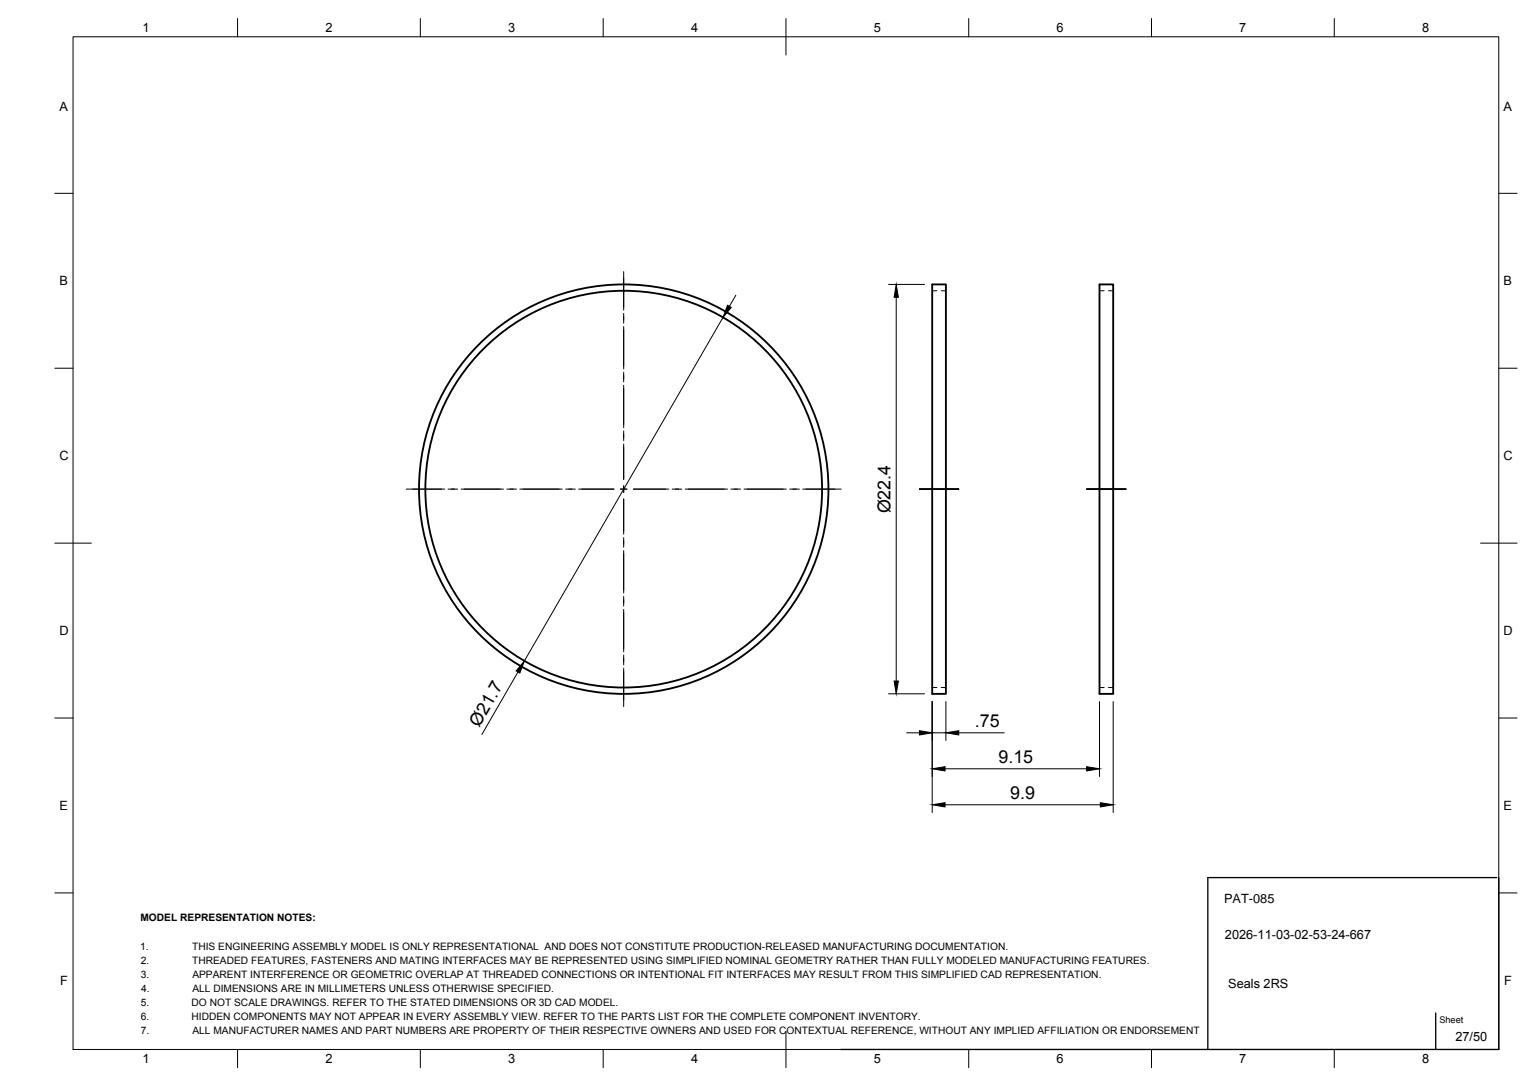
ISO-10303-21;
HEADER;
/* Generated by software containing ST-Developer
 * from STEP Tools, Inc. (www.steptools.com) 
 */

FILE_DESCRIPTION(
/* description */ ('Rack and pinion manual slide'),
/* implementation_level */ '2;1');

FILE_NAME(
/* name */ 'Seals 2RS.step',
/* time_stamp */ '2026-10-28T03:22:49-07:00',
/* author */ (''),
/* organization */ (''),
/* preprocessor_version */ 'ST-DEVELOPER v20.2',
/* originating_system */ 'Autodesk Translation Framework v15.17.0.0',
/* authorisation */ '');

FILE_SCHEMA (('AUTOMOTIVE_DESIGN { 1 0 10303 214 3 1 1 }'));
ENDSEC;

DATA;
#10=MECHANICAL_DESIGN_GEOMETRIC_PRESENTATION_REPRESENTATION('',(#761,#762),#34851);
#663=SHAPE_REPRESENTATION_RELATIONSHIP('SRR','None',#35099,#709);
#709=ADVANCED_BREP_SHAPE_REPRESENTATION('',(#813,#814),#34824);
#761=STYLED_ITEM('',(#35411),#813);
#762=STYLED_ITEM('',(#35411),#814);
#813=MANIFOLD_SOLID_BREP('Body1',#13782);
#814=MANIFOLD_SOLID_BREP('Body2',#13783);
#980=FACE_BOUND('',#2725,.T.);
#981=FACE_BOUND('',#2728,.T.);
#982=FACE_BOUND('',#2731,.T.);
#983=FACE_BOUND('',#2734,.T.);
#1230=PLANE('',#14885);
#1231=PLANE('',#14890);
#1232=PLANE('',#14893);
#1233=PLANE('',#14898);
#1838=FACE_OUTER_BOUND('',#2724,.T.);
#1839=FACE_OUTER_BOUND('',#2726,.T.);
#1840=FACE_OUTER_BOUND('',#2727,.T.);
#1841=FACE_OUTER_BOUND('',#2729,.T.);
#1842=FACE_OUTER_BOUND('',#2730,.T.);
#1843=FACE_OUTER_BOUND('',#2732,.T.);
#1844=FACE_OUTER_BOUND('',#2733,.T.);
#1845=FACE_OUTER_BOUND('',#2735,.T.);
#2724=EDGE_LOOP('',(#10664));
#2725=EDGE_LOOP('',(#10665));
#2726=EDGE_LOOP('',(#10666,#10667,#10668,#10669));
#2727=EDGE_LOOP('',(#10670));
#2728=EDGE_LOOP('',(#10671));
#2729=EDGE_LOOP('',(#10672,#10673,#10674,#10675));
#2730=EDGE_LOOP('',(#10676));
#2731=EDGE_LOOP('',(#10677));
#2732=EDGE_LOOP('',(#10678,#10679,#10680,#10681));
#2733=EDGE_LOOP('',(#10682));
#2734=EDGE_LOOP('',(#10683));
#2735=EDGE_LOOP('',(#10684,#10685,#10686,#10687));
#3687=LINE('',#21287,#4978);
#3688=LINE('',#21292,#4979);
#3689=LINE('',#21301,#4980);
#3690=LINE('',#21306,#4981);
#4978=VECTOR('',#17209,1.119765);
#4979=VECTOR('',#17216,1.085235);
#4980=VECTOR('',#17227,1.119765);
#4981=VECTOR('',#17234,1.085235);
#6042=CIRCLE('',#14886,1.119765);
#6043=CIRCLE('',#14887,1.085235);
#6044=CIRCLE('',#14889,1.119765);
#6045=CIRCLE('',#14891,1.085235);
#6046=CIRCLE('',#14894,1.119765);
#6047=CIRCLE('',#14895,1.085235);
#6048=CIRCLE('',#14897,1.119765);
#6049=CIRCLE('',#14899,1.085235);
#6707=VERTEX_POINT('',#21280);
#6708=VERTEX_POINT('',#21282);
#6709=VERTEX_POINT('',#21285);
#6710=VERTEX_POINT('',#21289);
#6711=VERTEX_POINT('',#21294);
#6712=VERTEX_POINT('',#21296);
#6713=VERTEX_POINT('',#21299);
#6714=VERTEX_POINT('',#21303);
#8144=EDGE_CURVE('',#6707,#6707,#6042,.T.);
#8145=EDGE_CURVE('',#6708,#6708,#6043,.T.);
#8146=EDGE_CURVE('',#6709,#6709,#6044,.T.);
#8147=EDGE_CURVE('',#6709,#6707,#3687,.T.);
#8148=EDGE_CURVE('',#6710,#6710,#6045,.T.);
#8149=EDGE_CURVE('',#6710,#6708,#3688,.T.);
#8150=EDGE_CURVE('',#6711,#6711,#6046,.T.);
#8151=EDGE_CURVE('',#6712,#6712,#6047,.T.);
#8152=EDGE_CURVE('',#6713,#6713,#6048,.T.);
#8153=EDGE_CURVE('',#6713,#6711,#3689,.T.);
#8154=EDGE_CURVE('',#6714,#6714,#6049,.T.);
#8155=EDGE_CURVE('',#6714,#6712,#3690,.T.);
#10664=ORIENTED_EDGE('',*,*,#8144,.F.);
#10665=ORIENTED_EDGE('',*,*,#8145,.T.);
#10666=ORIENTED_EDGE('',*,*,#8146,.F.);
#10667=ORIENTED_EDGE('',*,*,#8147,.T.);
#10668=ORIENTED_EDGE('',*,*,#8144,.T.);
#10669=ORIENTED_EDGE('',*,*,#8147,.F.);
#10670=ORIENTED_EDGE('',*,*,#8146,.T.);
#10671=ORIENTED_EDGE('',*,*,#8148,.F.);
#10672=ORIENTED_EDGE('',*,*,#8148,.T.);
#10673=ORIENTED_EDGE('',*,*,#8149,.T.);
#10674=ORIENTED_EDGE('',*,*,#8145,.F.);
#10675=ORIENTED_EDGE('',*,*,#8149,.F.);
#10676=ORIENTED_EDGE('',*,*,#8150,.F.);
#10677=ORIENTED_EDGE('',*,*,#8151,.T.);
#10678=ORIENTED_EDGE('',*,*,#8152,.F.);
#10679=ORIENTED_EDGE('',*,*,#8153,.T.);
#10680=ORIENTED_EDGE('',*,*,#8150,.T.);
#10681=ORIENTED_EDGE('',*,*,#8153,.F.);
#10682=ORIENTED_EDGE('',*,*,#8152,.T.);
#10683=ORIENTED_EDGE('',*,*,#8154,.F.);
#10684=ORIENTED_EDGE('',*,*,#8154,.T.);
#10685=ORIENTED_EDGE('',*,*,#8155,.T.);
#10686=ORIENTED_EDGE('',*,*,#8151,.F.);
#10687=ORIENTED_EDGE('',*,*,#8155,.F.);
#12936=CYLINDRICAL_SURFACE('',#14888,1.119765);
#12937=CYLINDRICAL_SURFACE('',#14892,1.085235);
#12938=CYLINDRICAL_SURFACE('',#14896,1.119765);
#12939=CYLINDRICAL_SURFACE('',#14900,1.085235);
#13316=ADVANCED_FACE('',(#1838,#980),#1230,.T.);
#13317=ADVANCED_FACE('',(#1839),#12936,.T.);
#13318=ADVANCED_FACE('',(#1840,#981),#1231,.T.);
#13319=ADVANCED_FACE('',(#1841),#12937,.F.);
#13320=ADVANCED_FACE('',(#1842,#982),#1232,.T.);
#13321=ADVANCED_FACE('',(#1843),#12938,.T.);
#13322=ADVANCED_FACE('',(#1844,#983),#1233,.T.);
#13323=ADVANCED_FACE('',(#1845),#12939,.F.);
#13782=CLOSED_SHELL('',(#13316,#13317,#13318,#13319));
#13783=CLOSED_SHELL('',(#13320,#13321,#13322,#13323));
#14884=AXIS2_PLACEMENT_3D('',#21278,#17197,#17198);
#14885=AXIS2_PLACEMENT_3D('',#21279,#17199,#17200);
#14886=AXIS2_PLACEMENT_3D('',#21281,#17201,#17202);
#14887=AXIS2_PLACEMENT_3D('',#21283,#17203,#17204);
#14888=AXIS2_PLACEMENT_3D('',#21284,#17205,#17206);
#14889=AXIS2_PLACEMENT_3D('',#21286,#17207,#17208);
#14890=AXIS2_PLACEMENT_3D('',#21288,#17210,#17211);
#14891=AXIS2_PLACEMENT_3D('',#21290,#17212,#17213);
#14892=AXIS2_PLACEMENT_3D('',#21291,#17214,#17215);
#14893=AXIS2_PLACEMENT_3D('',#21293,#17217,#17218);
#14894=AXIS2_PLACEMENT_3D('',#21295,#17219,#17220);
#14895=AXIS2_PLACEMENT_3D('',#21297,#17221,#17222);
#14896=AXIS2_PLACEMENT_3D('',#21298,#17223,#17224);
#14897=AXIS2_PLACEMENT_3D('',#21300,#17225,#17226);
#14898=AXIS2_PLACEMENT_3D('',#21302,#17228,#17229);
#14899=AXIS2_PLACEMENT_3D('',#21304,#17230,#17231);
#14900=AXIS2_PLACEMENT_3D('',#21305,#17232,#17233);
#17197=DIRECTION('axis',(0.,0.,1.));
#17198=DIRECTION('refdir',(1.,0.,0.));
#17199=DIRECTION('center_axis',(0.,1.,0.));
#17200=DIRECTION('ref_axis',(0.,0.,1.));
#17201=DIRECTION('center_axis',(0.,-1.,0.));
#17202=DIRECTION('ref_axis',(1.,0.,0.));
#17203=DIRECTION('center_axis',(0.,-1.,0.));
#17204=DIRECTION('ref_axis',(1.,0.,0.));
#17205=DIRECTION('center_axis',(0.,-1.,0.));
#17206=DIRECTION('ref_axis',(1.,0.,0.));
#17207=DIRECTION('center_axis',(0.,-1.,0.));
#17208=DIRECTION('ref_axis',(1.,0.,0.));
#17209=DIRECTION('',(0.,1.,0.));
#17210=DIRECTION('center_axis',(0.,-1.,0.));
#17211=DIRECTION('ref_axis',(0.,0.,-1.));
#17212=DIRECTION('center_axis',(0.,-1.,0.));
#17213=DIRECTION('ref_axis',(1.,0.,0.));
#17214=DIRECTION('center_axis',(0.,-1.,0.));
#17215=DIRECTION('ref_axis',(1.,0.,0.));
#17216=DIRECTION('',(0.,1.,0.));
#17217=DIRECTION('center_axis',(0.,1.,0.));
#17218=DIRECTION('ref_axis',(0.,0.,1.));
#17219=DIRECTION('center_axis',(0.,-1.,0.));
#17220=DIRECTION('ref_axis',(1.,0.,0.));
#17221=DIRECTION('center_axis',(0.,-1.,0.));
#17222=DIRECTION('ref_axis',(1.,0.,0.));
#17223=DIRECTION('center_axis',(0.,-1.,0.));
#17224=DIRECTION('ref_axis',(1.,0.,0.));
#17225=DIRECTION('center_axis',(0.,-1.,0.));
#17226=DIRECTION('ref_axis',(1.,0.,0.));
#17227=DIRECTION('',(0.,1.,0.));
#17228=DIRECTION('center_axis',(0.,-1.,0.));
#17229=DIRECTION('ref_axis',(0.,0.,-1.));
#17230=DIRECTION('center_axis',(0.,-1.,0.));
#17231=DIRECTION('ref_axis',(1.,0.,0.));
#17232=DIRECTION('center_axis',(0.,-1.,0.));
#17233=DIRECTION('ref_axis',(1.,0.,0.));
#17234=DIRECTION('',(0.,1.,0.));
#21278=CARTESIAN_POINT('',(0.,0.,0.));
#21279=CARTESIAN_POINT('Origin',(1.119765,0.495,0.));
#21280=CARTESIAN_POINT('',(-1.119765,0.495,-1.37131662304724E-16));
#21281=CARTESIAN_POINT('Origin',(0.,0.495,0.));
#21282=CARTESIAN_POINT('',(-1.085235,0.495,-1.32902956907268E-16));
#21283=CARTESIAN_POINT('Origin',(0.,0.495,0.));
#21284=CARTESIAN_POINT('Origin',(0.,0.4575,0.));
#21285=CARTESIAN_POINT('',(-1.119765,0.42,-1.37131662304724E-16));
#21286=CARTESIAN_POINT('Origin',(0.,0.42,0.));
#21287=CARTESIAN_POINT('',(-1.119765,0.4575,-1.37131662304724E-16));
#21288=CARTESIAN_POINT('Origin',(1.085235,0.42,0.));
#21289=CARTESIAN_POINT('',(-1.085235,0.42,-1.32902956907268E-16));
#21290=CARTESIAN_POINT('Origin',(0.,0.42,0.));
#21291=CARTESIAN_POINT('Origin',(0.,0.4575,0.));
#21292=CARTESIAN_POINT('',(-1.085235,0.4575,-1.32902956907268E-16));
#21293=CARTESIAN_POINT('Origin',(1.119765,-0.42,0.));
#21294=CARTESIAN_POINT('',(-1.119765,-0.42,-1.37131662304724E-16));
#21295=CARTESIAN_POINT('Origin',(0.,-0.42,0.));
#21296=CARTESIAN_POINT('',(-1.085235,-0.42,-1.32902956907268E-16));
#21297=CARTESIAN_POINT('Origin',(0.,-0.42,0.));
#21298=CARTESIAN_POINT('Origin',(0.,-0.4575,0.));
#21299=CARTESIAN_POINT('',(-1.119765,-0.495,-1.37131662304724E-16));
#21300=CARTESIAN_POINT('Origin',(0.,-0.495,0.));
#21301=CARTESIAN_POINT('',(-1.119765,-0.4575,-1.37131662304724E-16));
#21302=CARTESIAN_POINT('Origin',(1.085235,-0.495,0.));
#21303=CARTESIAN_POINT('',(-1.085235,-0.495,-1.32902956907268E-16));
#21304=CARTESIAN_POINT('Origin',(0.,-0.495,0.));
#21305=CARTESIAN_POINT('Origin',(0.,-0.4575,0.));
#21306=CARTESIAN_POINT('',(-1.085235,-0.4575,-1.32902956907268E-16));
#34770=UNCERTAINTY_MEASURE_WITH_UNIT(LENGTH_MEASURE(0.001),#34852,
'DISTANCE_ACCURACY_VALUE',
'Maximum model space distance between geometric entities at asserted c
onnectivities');
#34797=UNCERTAINTY_MEASURE_WITH_UNIT(LENGTH_MEASURE(0.001),#34852,
'DISTANCE_ACCURACY_VALUE',
'Maximum model space distance between geometric entities at asserted c
onnectivities');
#34824=(
GEOMETRIC_REPRESENTATION_CONTEXT(3)
GLOBAL_UNCERTAINTY_ASSIGNED_CONTEXT((#34770))
GLOBAL_UNIT_ASSIGNED_CONTEXT((#34852,#34854,#34855))
REPRESENTATION_CONTEXT('','3D')
);
#34851=(
GEOMETRIC_REPRESENTATION_CONTEXT(3)
GLOBAL_UNCERTAINTY_ASSIGNED_CONTEXT((#34797))
GLOBAL_UNIT_ASSIGNED_CONTEXT((#34852,#34854,#34855))
REPRESENTATION_CONTEXT('','3D')
);
#34852=(
LENGTH_UNIT()
NAMED_UNIT(*)
SI_UNIT(.CENTI.,.METRE.)
);
#34854=(
NAMED_UNIT(*)
PLANE_ANGLE_UNIT()
SI_UNIT($,.RADIAN.)
);
#34855=(
NAMED_UNIT(*)
SI_UNIT($,.STERADIAN.)
SOLID_ANGLE_UNIT()
);
#34882=SHAPE_DEFINITION_REPRESENTATION(#34935,#35099);
#34935=PRODUCT_DEFINITION_SHAPE('',$,#35153);
#35099=SHAPE_REPRESENTATION('',(#14884),#34824);
#35126=PRODUCT_DEFINITION_CONTEXT('part definition',#35287,'design');
#35153=PRODUCT_DEFINITION('Seals 2RS','Seals 2RS',#35206,#35126);
#35206=PRODUCT_DEFINITION_FORMATION('',$,#35315);
#35287=APPLICATION_CONTEXT(
'Core Data for Automotive Mechanical Design Process');
#35288=PRODUCT_CONTEXT('part definition',#35287,'mechanical');
#35315=PRODUCT('Seals 2RS','Seals 2RS','Seals 2RS',(#35288));
#35405=COLOUR_RGB('Grey',0.48,0.52,0.57);
#35406=FILL_AREA_STYLE_COLOUR('',#35405);
#35407=FILL_AREA_STYLE('',(#35406));
#35408=SURFACE_STYLE_FILL_AREA(#35407);
#35409=SURFACE_SIDE_STYLE('',(#35408));
#35410=SURFACE_STYLE_USAGE(.BOTH.,#35409);
#35411=PRESENTATION_STYLE_ASSIGNMENT((#35410));
ENDSEC;
END-ISO-10303-21;
